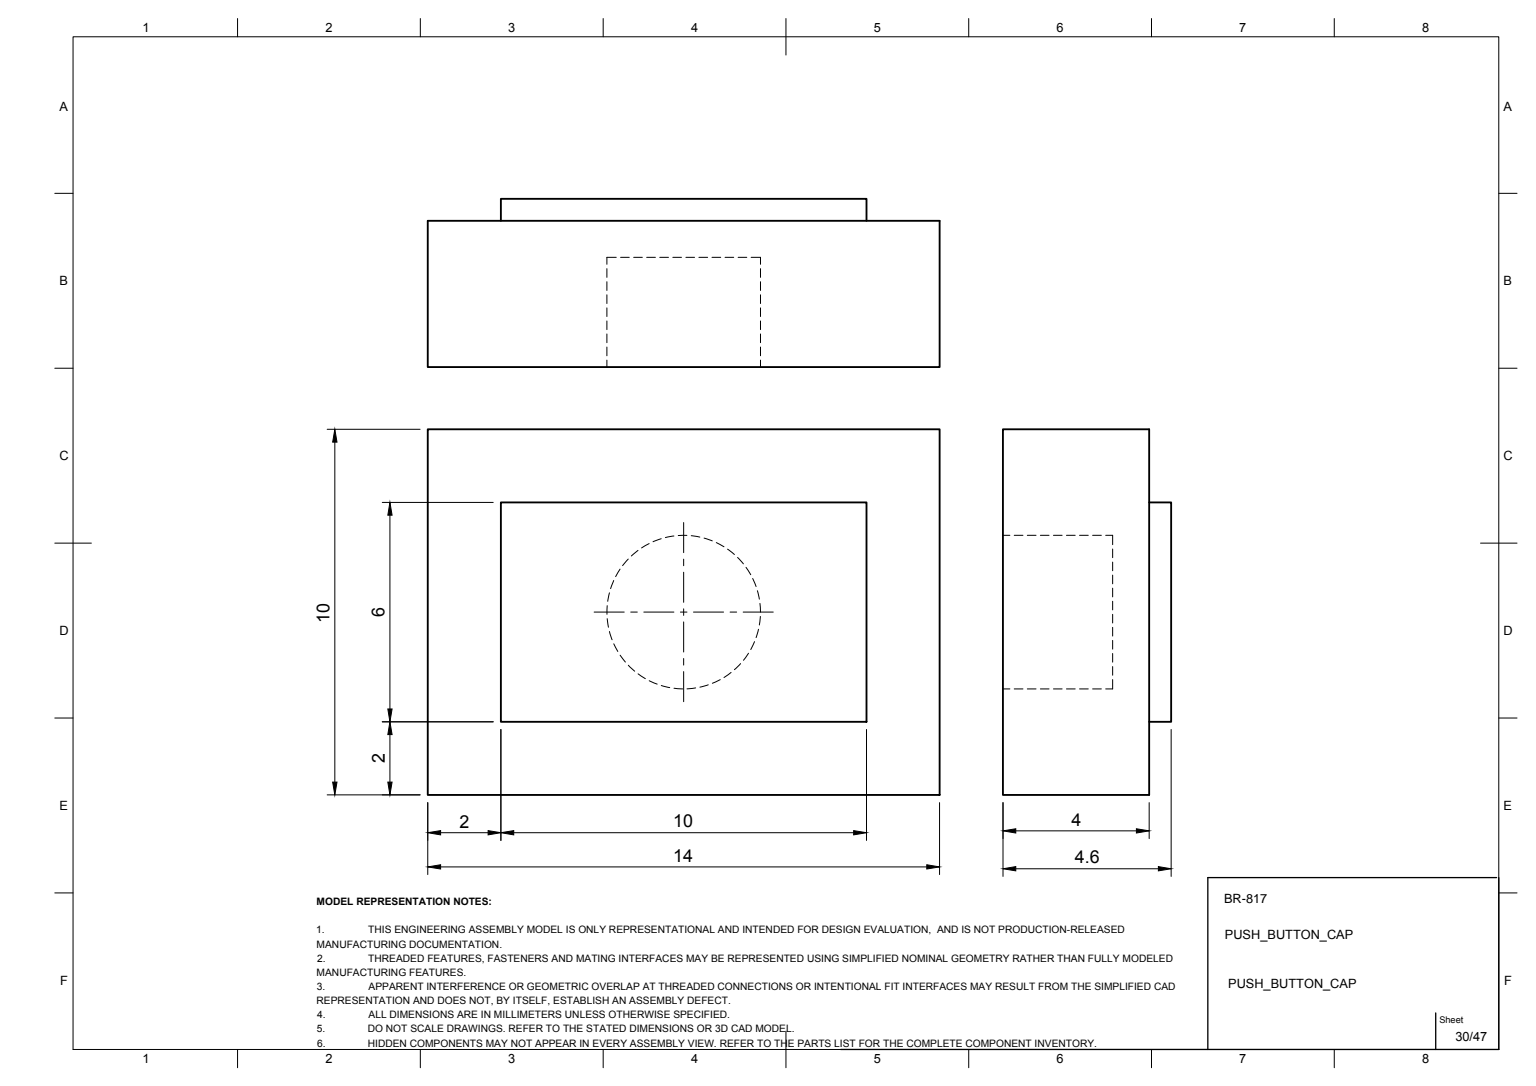
ISO-10303-21;
HEADER;
FILE_DESCRIPTION((''),'2;1');
FILE_NAME('PUSH_BUTTON_CAP.step','2026-10-01T22:07:29-07:00',(''),(''),'','','');
FILE_SCHEMA (('AUTOMOTIVE_DESIGN { 1 0 10303 214 3 1 1 }'));
ENDSEC;
DATA;
#10=MECHANICAL_DESIGN_GEOMETRIC_PRESENTATION_REPRESENTATION('',(#562),#15484);
#492=SHAPE_REPRESENTATION_RELATIONSHIP('SRR','None',#15642,#527) ;
#527=ADVANCED_BREP_SHAPE_REPRESENTATION('',(#603),#15466) ;
#562=STYLED_ITEM('',(#15838),#603) ;
#603=MANIFOLD_SOLID_BREP('PUSH_BUTTON_CAP',#8273) ;
#731=CYLINDRICAL_SURFACE('',#9339,0.21) ;
#873=FACE_BOUND('',#2213,.T.) ;
#874=FACE_BOUND('',#2215,.T.) ;
#1145=CIRCLE('',#9340,0.21) ;
#1146=CIRCLE('',#9341,0.21) ;
#1642=FACE_OUTER_BOUND('',#2205,.T.) ;
#1643=FACE_OUTER_BOUND('',#2206,.T.) ;
#1644=FACE_OUTER_BOUND('',#2207,.T.) ;
#1645=FACE_OUTER_BOUND('',#2208,.T.) ;
#1646=FACE_OUTER_BOUND('',#2209,.T.) ;
#1647=FACE_OUTER_BOUND('',#2210,.T.) ;
#1648=FACE_OUTER_BOUND('',#2211,.T.) ;
#1649=FACE_OUTER_BOUND('',#2212,.T.) ;
#1650=FACE_OUTER_BOUND('',#2214,.T.) ;
#1651=FACE_OUTER_BOUND('',#2216,.T.) ;
#1652=FACE_OUTER_BOUND('',#2217,.T.) ;
#1653=FACE_OUTER_BOUND('',#2218,.T.) ;
#1654=FACE_OUTER_BOUND('',#2219,.T.) ;
#2205=EDGE_LOOP('',(#6511,#6512,#6513,#6514)) ;
#2206=EDGE_LOOP('',(#6515,#6516,#6517,#6518)) ;
#2207=EDGE_LOOP('',(#6519,#6520,#6521,#6522)) ;
#2208=EDGE_LOOP('',(#6523,#6524,#6525,#6526)) ;
#2209=EDGE_LOOP('',(#6527,#6528,#6529,#6530)) ;
#2210=EDGE_LOOP('',(#6531,#6532,#6533,#6534)) ;
#2211=EDGE_LOOP('',(#6535)) ;
#2212=EDGE_LOOP('',(#6536,#6537,#6538,#6539)) ;
#2213=EDGE_LOOP('',(#6540,#6541,#6542,#6543)) ;
#2214=EDGE_LOOP('',(#6544,#6545,#6546,#6547)) ;
#2215=EDGE_LOOP('',(#6548)) ;
#2216=EDGE_LOOP('',(#6549,#6550,#6551,#6552)) ;
#2217=EDGE_LOOP('',(#6553,#6554,#6555,#6556)) ;
#2218=EDGE_LOOP('',(#6557,#6558,#6559,#6560)) ;
#2219=EDGE_LOOP('',(#6561,#6562,#6563,#6564)) ;
#2722=LINE('',#14279,#3196) ;
#2723=LINE('',#14281,#3197) ;
#2724=LINE('',#14283,#3198) ;
#2725=LINE('',#14284,#3199) ;
#2726=LINE('',#14287,#3200) ;
#2727=LINE('',#14289,#3201) ;
#2728=LINE('',#14290,#3202) ;
#2729=LINE('',#14293,#3203) ;
#2730=LINE('',#14294,#3204) ;
#2731=LINE('',#14297,#3205) ;
#2732=LINE('',#14298,#3206) ;
#2733=LINE('',#14300,#3207) ;
#2734=LINE('',#14305,#3208) ;
#2735=LINE('',#14311,#3209) ;
#2736=LINE('',#14313,#3210) ;
#2737=LINE('',#14315,#3211) ;
#2738=LINE('',#14316,#3212) ;
#2739=LINE('',#14320,#3213) ;
#2740=LINE('',#14322,#3214) ;
#2741=LINE('',#14324,#3215) ;
#2742=LINE('',#14325,#3216) ;
#2743=LINE('',#14327,#3217) ;
#2744=LINE('',#14328,#3218) ;
#2745=LINE('',#14330,#3219) ;
#2746=LINE('',#14332,#3220) ;
#3196=VECTOR('',#11513,1.) ;
#3197=VECTOR('',#11514,1.) ;
#3198=VECTOR('',#11515,1.) ;
#3199=VECTOR('',#11516,1.) ;
#3200=VECTOR('',#11519,1.) ;
#3201=VECTOR('',#11520,1.) ;
#3202=VECTOR('',#11521,1.) ;
#3203=VECTOR('',#11524,1.) ;
#3204=VECTOR('',#11525,1.) ;
#3205=VECTOR('',#11528,1.) ;
#3206=VECTOR('',#11529,1.) ;
#3207=VECTOR('',#11532,1.) ;
#3208=VECTOR('',#11537,0.21) ;
#3209=VECTOR('',#11544,1.) ;
#3210=VECTOR('',#11545,1.) ;
#3211=VECTOR('',#11546,1.) ;
#3212=VECTOR('',#11547,1.) ;
#3213=VECTOR('',#11550,1.) ;
#3214=VECTOR('',#11551,1.) ;
#3215=VECTOR('',#11552,1.) ;
#3216=VECTOR('',#11553,1.) ;
#3217=VECTOR('',#11556,1.) ;
#3218=VECTOR('',#11557,1.) ;
#3219=VECTOR('',#11560,1.) ;
#3220=VECTOR('',#11563,1.) ;
#3801=VERTEX_POINT('',#14277) ;
#3802=VERTEX_POINT('',#14278) ;
#3803=VERTEX_POINT('',#14280) ;
#3804=VERTEX_POINT('',#14282) ;
#3805=VERTEX_POINT('',#14286) ;
#3806=VERTEX_POINT('',#14288) ;
#3807=VERTEX_POINT('',#14292) ;
#3808=VERTEX_POINT('',#14296) ;
#3809=VERTEX_POINT('',#14302) ;
#3810=VERTEX_POINT('',#14304) ;
#3811=VERTEX_POINT('',#14309) ;
#3812=VERTEX_POINT('',#14310) ;
#3813=VERTEX_POINT('',#14312) ;
#3814=VERTEX_POINT('',#14314) ;
#3815=VERTEX_POINT('',#14318) ;
#3816=VERTEX_POINT('',#14319) ;
#3817=VERTEX_POINT('',#14321) ;
#3818=VERTEX_POINT('',#14323) ;
#4760=EDGE_CURVE('',#3801,#3802,#2722,.T.) ;
#4761=EDGE_CURVE('',#3802,#3803,#2723,.T.) ;
#4762=EDGE_CURVE('',#3803,#3804,#2724,.T.) ;
#4763=EDGE_CURVE('',#3804,#3801,#2725,.T.) ;
#4764=EDGE_CURVE('',#3804,#3805,#2726,.T.) ;
#4765=EDGE_CURVE('',#3806,#3805,#2727,.T.) ;
#4766=EDGE_CURVE('',#3801,#3806,#2728,.T.) ;
#4767=EDGE_CURVE('',#3803,#3807,#2729,.T.) ;
#4768=EDGE_CURVE('',#3805,#3807,#2730,.T.) ;
#4769=EDGE_CURVE('',#3802,#3808,#2731,.T.) ;
#4770=EDGE_CURVE('',#3807,#3808,#2732,.T.) ;
#4771=EDGE_CURVE('',#3808,#3806,#2733,.T.) ;
#4772=EDGE_CURVE('',#3809,#3809,#1145,.T.) ;
#4773=EDGE_CURVE('',#3809,#3810,#2734,.T.) ;
#4774=EDGE_CURVE('',#3810,#3810,#1146,.T.) ;
#4775=EDGE_CURVE('',#3811,#3812,#2735,.T.) ;
#4776=EDGE_CURVE('',#3812,#3813,#2736,.T.) ;
#4777=EDGE_CURVE('',#3813,#3814,#2737,.T.) ;
#4778=EDGE_CURVE('',#3814,#3811,#2738,.T.) ;
#4779=EDGE_CURVE('',#3815,#3816,#2739,.T.) ;
#4780=EDGE_CURVE('',#3816,#3817,#2740,.T.) ;
#4781=EDGE_CURVE('',#3817,#3818,#2741,.T.) ;
#4782=EDGE_CURVE('',#3818,#3815,#2742,.T.) ;
#4783=EDGE_CURVE('',#3814,#3817,#2743,.T.) ;
#4784=EDGE_CURVE('',#3811,#3816,#2744,.T.) ;
#4785=EDGE_CURVE('',#3813,#3818,#2745,.T.) ;
#4786=EDGE_CURVE('',#3812,#3815,#2746,.T.) ;
#6511=ORIENTED_EDGE('',*,*,#4760,.T.) ;
#6512=ORIENTED_EDGE('',*,*,#4761,.T.) ;
#6513=ORIENTED_EDGE('',*,*,#4762,.T.) ;
#6514=ORIENTED_EDGE('',*,*,#4763,.T.) ;
#6515=ORIENTED_EDGE('',*,*,#4764,.T.) ;
#6516=ORIENTED_EDGE('',*,*,#4765,.F.) ;
#6517=ORIENTED_EDGE('',*,*,#4766,.F.) ;
#6518=ORIENTED_EDGE('',*,*,#4763,.F.) ;
#6519=ORIENTED_EDGE('',*,*,#4767,.T.) ;
#6520=ORIENTED_EDGE('',*,*,#4768,.F.) ;
#6521=ORIENTED_EDGE('',*,*,#4764,.F.) ;
#6522=ORIENTED_EDGE('',*,*,#4762,.F.) ;
#6523=ORIENTED_EDGE('',*,*,#4769,.T.) ;
#6524=ORIENTED_EDGE('',*,*,#4770,.F.) ;
#6525=ORIENTED_EDGE('',*,*,#4767,.F.) ;
#6526=ORIENTED_EDGE('',*,*,#4761,.F.) ;
#6527=ORIENTED_EDGE('',*,*,#4766,.T.) ;
#6528=ORIENTED_EDGE('',*,*,#4771,.F.) ;
#6529=ORIENTED_EDGE('',*,*,#4769,.F.) ;
#6530=ORIENTED_EDGE('',*,*,#4760,.F.) ;
#6531=ORIENTED_EDGE('',*,*,#4772,.F.) ;
#6532=ORIENTED_EDGE('',*,*,#4773,.T.) ;
#6533=ORIENTED_EDGE('',*,*,#4774,.T.) ;
#6534=ORIENTED_EDGE('',*,*,#4773,.F.) ;
#6535=ORIENTED_EDGE('',*,*,#4774,.F.) ;
#6536=ORIENTED_EDGE('',*,*,#4775,.T.) ;
#6537=ORIENTED_EDGE('',*,*,#4776,.T.) ;
#6538=ORIENTED_EDGE('',*,*,#4777,.T.) ;
#6539=ORIENTED_EDGE('',*,*,#4778,.T.) ;
#6540=ORIENTED_EDGE('',*,*,#4765,.T.) ;
#6541=ORIENTED_EDGE('',*,*,#4768,.T.) ;
#6542=ORIENTED_EDGE('',*,*,#4770,.T.) ;
#6543=ORIENTED_EDGE('',*,*,#4771,.T.) ;
#6544=ORIENTED_EDGE('',*,*,#4779,.T.) ;
#6545=ORIENTED_EDGE('',*,*,#4780,.T.) ;
#6546=ORIENTED_EDGE('',*,*,#4781,.T.) ;
#6547=ORIENTED_EDGE('',*,*,#4782,.T.) ;
#6548=ORIENTED_EDGE('',*,*,#4772,.T.) ;
#6549=ORIENTED_EDGE('',*,*,#4783,.T.) ;
#6550=ORIENTED_EDGE('',*,*,#4780,.F.) ;
#6551=ORIENTED_EDGE('',*,*,#4784,.F.) ;
#6552=ORIENTED_EDGE('',*,*,#4778,.F.) ;
#6553=ORIENTED_EDGE('',*,*,#4785,.T.) ;
#6554=ORIENTED_EDGE('',*,*,#4781,.F.) ;
#6555=ORIENTED_EDGE('',*,*,#4783,.F.) ;
#6556=ORIENTED_EDGE('',*,*,#4777,.F.) ;
#6557=ORIENTED_EDGE('',*,*,#4786,.T.) ;
#6558=ORIENTED_EDGE('',*,*,#4782,.F.) ;
#6559=ORIENTED_EDGE('',*,*,#4785,.F.) ;
#6560=ORIENTED_EDGE('',*,*,#4776,.F.) ;
#6561=ORIENTED_EDGE('',*,*,#4784,.T.) ;
#6562=ORIENTED_EDGE('',*,*,#4779,.F.) ;
#6563=ORIENTED_EDGE('',*,*,#4786,.F.) ;
#6564=ORIENTED_EDGE('',*,*,#4775,.F.) ;
#7664=PLANE('',#9334) ;
#7665=PLANE('',#9335) ;
#7666=PLANE('',#9336) ;
#7667=PLANE('',#9337) ;
#7668=PLANE('',#9338) ;
#7669=PLANE('',#9342) ;
#7670=PLANE('',#9343) ;
#7671=PLANE('',#9344) ;
#7672=PLANE('',#9345) ;
#7673=PLANE('',#9346) ;
#7674=PLANE('',#9347) ;
#7675=PLANE('',#9348) ;
#8029=ADVANCED_FACE('',(#1642),#7664,.T.) ;
#8030=ADVANCED_FACE('',(#1643),#7665,.F.) ;
#8031=ADVANCED_FACE('',(#1644),#7666,.F.) ;
#8032=ADVANCED_FACE('',(#1645),#7667,.F.) ;
#8033=ADVANCED_FACE('',(#1646),#7668,.F.) ;
#8034=ADVANCED_FACE('',(#1647),#731,.F.) ;
#8035=ADVANCED_FACE('',(#1648),#7669,.F.) ;
#8036=ADVANCED_FACE('',(#1649,#873),#7670,.T.) ;
#8037=ADVANCED_FACE('',(#1650,#874),#7671,.F.) ;
#8038=ADVANCED_FACE('',(#1651),#7672,.F.) ;
#8039=ADVANCED_FACE('',(#1652),#7673,.F.) ;
#8040=ADVANCED_FACE('',(#1653),#7674,.F.) ;
#8041=ADVANCED_FACE('',(#1654),#7675,.F.) ;
#8273=CLOSED_SHELL('',(#8029,#8030,#8031,#8032,#8033,#8034,#8035,#8036,
#8037,#8038,#8039,#8040,#8041)) ;
#9333=AXIS2_PLACEMENT_3D('',#14275,#11509,#11510) ;
#9334=AXIS2_PLACEMENT_3D('',#14276,#11511,#11512) ;
#9335=AXIS2_PLACEMENT_3D('',#14285,#11517,#11518) ;
#9336=AXIS2_PLACEMENT_3D('',#14291,#11522,#11523) ;
#9337=AXIS2_PLACEMENT_3D('',#14295,#11526,#11527) ;
#9338=AXIS2_PLACEMENT_3D('',#14299,#11530,#11531) ;
#9339=AXIS2_PLACEMENT_3D('',#14301,#11533,#11534) ;
#9340=AXIS2_PLACEMENT_3D('',#14303,#11535,#11536) ;
#9341=AXIS2_PLACEMENT_3D('',#14306,#11538,#11539) ;
#9342=AXIS2_PLACEMENT_3D('',#14307,#11540,#11541) ;
#9343=AXIS2_PLACEMENT_3D('',#14308,#11542,#11543) ;
#9344=AXIS2_PLACEMENT_3D('',#14317,#11548,#11549) ;
#9345=AXIS2_PLACEMENT_3D('',#14326,#11554,#11555) ;
#9346=AXIS2_PLACEMENT_3D('',#14329,#11558,#11559) ;
#9347=AXIS2_PLACEMENT_3D('',#14331,#11561,#11562) ;
#9348=AXIS2_PLACEMENT_3D('',#14333,#11564,#11565) ;
#11509=DIRECTION('axis',(0.,0.,1.)) ;
#11510=DIRECTION('refdir',(1.,0.,0.)) ;
#11511=DIRECTION('center_axis',(0.,0.,1.)) ;
#11512=DIRECTION('ref_axis',(1.,0.,0.)) ;
#11513=DIRECTION('',(0.,1.,0.)) ;
#11514=DIRECTION('',(-1.,0.,0.)) ;
#11515=DIRECTION('',(0.,-1.,0.)) ;
#11516=DIRECTION('',(1.,0.,0.)) ;
#11517=DIRECTION('center_axis',(0.,1.,0.)) ;
#11518=DIRECTION('ref_axis',(0.,0.,1.)) ;
#11519=DIRECTION('',(0.,0.,-1.)) ;
#11520=DIRECTION('',(-1.,0.,0.)) ;
#11521=DIRECTION('',(0.,0.,-1.)) ;
#11522=DIRECTION('center_axis',(1.,0.,0.)) ;
#11523=DIRECTION('ref_axis',(0.,0.,-1.)) ;
#11524=DIRECTION('',(0.,0.,-1.)) ;
#11525=DIRECTION('',(0.,1.,0.)) ;
#11526=DIRECTION('center_axis',(0.,-1.,0.)) ;
#11527=DIRECTION('ref_axis',(0.,0.,-1.)) ;
#11528=DIRECTION('',(0.,0.,-1.)) ;
#11529=DIRECTION('',(1.,0.,0.)) ;
#11530=DIRECTION('center_axis',(-1.,0.,0.)) ;
#11531=DIRECTION('ref_axis',(0.,0.,1.)) ;
#11532=DIRECTION('',(0.,-1.,0.)) ;
#11533=DIRECTION('center_axis',(0.,0.,1.)) ;
#11534=DIRECTION('ref_axis',(1.,0.,0.)) ;
#11535=DIRECTION('center_axis',(0.,0.,1.)) ;
#11536=DIRECTION('ref_axis',(1.,0.,0.)) ;
#11537=DIRECTION('',(0.,0.,1.)) ;
#11538=DIRECTION('center_axis',(0.,0.,1.)) ;
#11539=DIRECTION('ref_axis',(1.,0.,0.)) ;
#11540=DIRECTION('center_axis',(0.,0.,1.)) ;
#11541=DIRECTION('ref_axis',(1.,0.,0.)) ;
#11542=DIRECTION('center_axis',(0.,0.,1.)) ;
#11543=DIRECTION('ref_axis',(1.,0.,0.)) ;
#11544=DIRECTION('',(0.,1.,0.)) ;
#11545=DIRECTION('',(-1.,0.,0.)) ;
#11546=DIRECTION('',(0.,-1.,0.)) ;
#11547=DIRECTION('',(1.,0.,0.)) ;
#11548=DIRECTION('center_axis',(0.,0.,1.)) ;
#11549=DIRECTION('ref_axis',(1.,0.,0.)) ;
#11550=DIRECTION('',(0.,-1.,0.)) ;
#11551=DIRECTION('',(-1.,0.,0.)) ;
#11552=DIRECTION('',(0.,1.,0.)) ;
#11553=DIRECTION('',(1.,0.,0.)) ;
#11554=DIRECTION('center_axis',(0.,1.,0.)) ;
#11555=DIRECTION('ref_axis',(0.,0.,1.)) ;
#11556=DIRECTION('',(0.,0.,-1.)) ;
#11557=DIRECTION('',(0.,0.,-1.)) ;
#11558=DIRECTION('center_axis',(1.,0.,0.)) ;
#11559=DIRECTION('ref_axis',(0.,0.,-1.)) ;
#11560=DIRECTION('',(0.,0.,-1.)) ;
#11561=DIRECTION('center_axis',(0.,-1.,0.)) ;
#11562=DIRECTION('ref_axis',(0.,0.,-1.)) ;
#11563=DIRECTION('',(0.,0.,-1.)) ;
#11564=DIRECTION('center_axis',(-1.,0.,0.)) ;
#11565=DIRECTION('ref_axis',(0.,0.,1.)) ;
#14275=CARTESIAN_POINT('',(0.,0.,0.)) ;
#14276=CARTESIAN_POINT('Origin',(-3.,1.8,2.86)) ;
#14277=CARTESIAN_POINT('',(-2.5,1.5,2.86)) ;
#14278=CARTESIAN_POINT('',(-2.5,2.1,2.86)) ;
#14279=CARTESIAN_POINT('',(-2.5,1.8,2.86)) ;
#14280=CARTESIAN_POINT('',(-3.5,2.1,2.86)) ;
#14281=CARTESIAN_POINT('',(-3.,2.1,2.86)) ;
#14282=CARTESIAN_POINT('',(-3.5,1.5,2.86)) ;
#14283=CARTESIAN_POINT('',(-3.5,1.8,2.86)) ;
#14284=CARTESIAN_POINT('',(-3.,1.5,2.86)) ;
#14285=CARTESIAN_POINT('Origin',(-3.,1.5,2.83)) ;
#14286=CARTESIAN_POINT('',(-3.5,1.5,2.8)) ;
#14287=CARTESIAN_POINT('',(-3.5,1.5,2.83)) ;
#14288=CARTESIAN_POINT('',(-2.5,1.5,2.8)) ;
#14289=CARTESIAN_POINT('',(-3.,1.5,2.8)) ;
#14290=CARTESIAN_POINT('',(-2.5,1.5,2.83)) ;
#14291=CARTESIAN_POINT('Origin',(-3.5,1.8,2.83)) ;
#14292=CARTESIAN_POINT('',(-3.5,2.1,2.8)) ;
#14293=CARTESIAN_POINT('',(-3.5,2.1,2.83)) ;
#14294=CARTESIAN_POINT('',(-3.5,1.8,2.8)) ;
#14295=CARTESIAN_POINT('Origin',(-3.,2.1,2.83)) ;
#14296=CARTESIAN_POINT('',(-2.5,2.1,2.8)) ;
#14297=CARTESIAN_POINT('',(-2.5,2.1,2.83)) ;
#14298=CARTESIAN_POINT('',(-3.,2.1,2.8)) ;
#14299=CARTESIAN_POINT('Origin',(-2.5,1.8,2.83)) ;
#14300=CARTESIAN_POINT('',(-2.5,1.8,2.8)) ;
#14301=CARTESIAN_POINT('Origin',(-3.,1.8,2.5)) ;
#14302=CARTESIAN_POINT('',(-3.21,1.8,2.4)) ;
#14303=CARTESIAN_POINT('Origin',(-3.,1.8,2.4)) ;
#14304=CARTESIAN_POINT('',(-3.21,1.8,2.7)) ;
#14305=CARTESIAN_POINT('',(-3.21,1.8,2.5)) ;
#14306=CARTESIAN_POINT('Origin',(-3.,1.8,2.7)) ;
#14307=CARTESIAN_POINT('Origin',(-3.,1.8,2.7)) ;
#14308=CARTESIAN_POINT('Origin',(-3.,1.8,2.8)) ;
#14309=CARTESIAN_POINT('',(-2.3,1.3,2.8)) ;
#14310=CARTESIAN_POINT('',(-2.3,2.3,2.8)) ;
#14311=CARTESIAN_POINT('',(-2.3,1.8,2.8)) ;
#14312=CARTESIAN_POINT('',(-3.7,2.3,2.8)) ;
#14313=CARTESIAN_POINT('',(-3.,2.3,2.8)) ;
#14314=CARTESIAN_POINT('',(-3.7,1.3,2.8)) ;
#14315=CARTESIAN_POINT('',(-3.7,1.8,2.8)) ;
#14316=CARTESIAN_POINT('',(-3.,1.3,2.8)) ;
#14317=CARTESIAN_POINT('Origin',(-3.,1.8,2.4)) ;
#14318=CARTESIAN_POINT('',(-2.3,2.3,2.4)) ;
#14319=CARTESIAN_POINT('',(-2.3,1.3,2.4)) ;
#14320=CARTESIAN_POINT('',(-2.3,1.8,2.4)) ;
#14321=CARTESIAN_POINT('',(-3.7,1.3,2.4)) ;
#14322=CARTESIAN_POINT('',(-3.,1.3,2.4)) ;
#14323=CARTESIAN_POINT('',(-3.7,2.3,2.4)) ;
#14324=CARTESIAN_POINT('',(-3.7,1.8,2.4)) ;
#14325=CARTESIAN_POINT('',(-3.,2.3,2.4)) ;
#14326=CARTESIAN_POINT('Origin',(-3.,1.3,2.6)) ;
#14327=CARTESIAN_POINT('',(-3.7,1.3,2.6)) ;
#14328=CARTESIAN_POINT('',(-2.3,1.3,2.6)) ;
#14329=CARTESIAN_POINT('Origin',(-3.7,1.8,2.6)) ;
#14330=CARTESIAN_POINT('',(-3.7,2.3,2.6)) ;
#14331=CARTESIAN_POINT('Origin',(-3.,2.3,2.6)) ;
#14332=CARTESIAN_POINT('',(-2.3,2.3,2.6)) ;
#14333=CARTESIAN_POINT('Origin',(-2.3,1.8,2.6)) ;
#15423=UNCERTAINTY_MEASURE_WITH_UNIT(LENGTH_MEASURE(0.001),#15485,
'DISTANCE_ACCURACY_VALUE',
'Maximum model space distance between geometric entities at asserted c
onnectivities') ;
#15441=UNCERTAINTY_MEASURE_WITH_UNIT(LENGTH_MEASURE(0.001),#15485,
'DISTANCE_ACCURACY_VALUE',
'Maximum model space distance between geometric entities at asserted c
onnectivities') ;
#15466=(
GEOMETRIC_REPRESENTATION_CONTEXT(3)
GLOBAL_UNCERTAINTY_ASSIGNED_CONTEXT((#15423))
GLOBAL_UNIT_ASSIGNED_CONTEXT((#15485,#15487,#15488))
REPRESENTATION_CONTEXT('','3D')
) ;
#15484=(
GEOMETRIC_REPRESENTATION_CONTEXT(3)
GLOBAL_UNCERTAINTY_ASSIGNED_CONTEXT((#15441))
GLOBAL_UNIT_ASSIGNED_CONTEXT((#15485,#15487,#15488))
REPRESENTATION_CONTEXT('','3D')
) ;
#15485=(
LENGTH_UNIT()
NAMED_UNIT(*)
SI_UNIT(.CENTI.,.METRE.)
) ;
#15487=(
NAMED_UNIT(*)
PLANE_ANGLE_UNIT()
SI_UNIT($,.RADIAN.)
) ;
#15488=(
NAMED_UNIT(*)
SI_UNIT($,.STERADIAN.)
SOLID_ANGLE_UNIT()
) ;
#15513=SHAPE_DEFINITION_REPRESENTATION(#15570,#15642) ;
#15570=PRODUCT_DEFINITION_SHAPE('',$,#15685) ;
#15642=SHAPE_REPRESENTATION('',(#9333),#15466) ;
#15660=PRODUCT_DEFINITION_CONTEXT('part definition',#15788,'design') ;
#15685=PRODUCT_DEFINITION('PUSH_BUTTON_CAP','PUSH_BUTTON_CAP',#15727,
#15660) ;
#15727=PRODUCT_DEFINITION_FORMATION('',$,#15814) ;
#15788=APPLICATION_CONTEXT(
'Core Data for Automotive Mechanical Design Process') ;
#15789=PRODUCT_CONTEXT('part definition',#15788,'mechanical') ;
#15814=PRODUCT('PUSH_BUTTON_CAP','PUSH_BUTTON_CAP',$,(#15789)) ;
#15838=PRESENTATION_STYLE_ASSIGNMENT((#15850)) ;
#15850=SURFACE_STYLE_USAGE(.BOTH.,#15862) ;
#15862=SURFACE_SIDE_STYLE('',(#15874)) ;
#15874=SURFACE_STYLE_FILL_AREA(#15886) ;
#15886=FILL_AREA_STYLE('ABS (White)',(#15898)) ;
#15898=FILL_AREA_STYLE_COLOUR('ABS (White)',#15910) ;
#15910=COLOUR_RGB('ABS (White)', 0.31764706, 0.68627451, 0.89019608) ;
ENDSEC;
END-ISO-10303-21;
